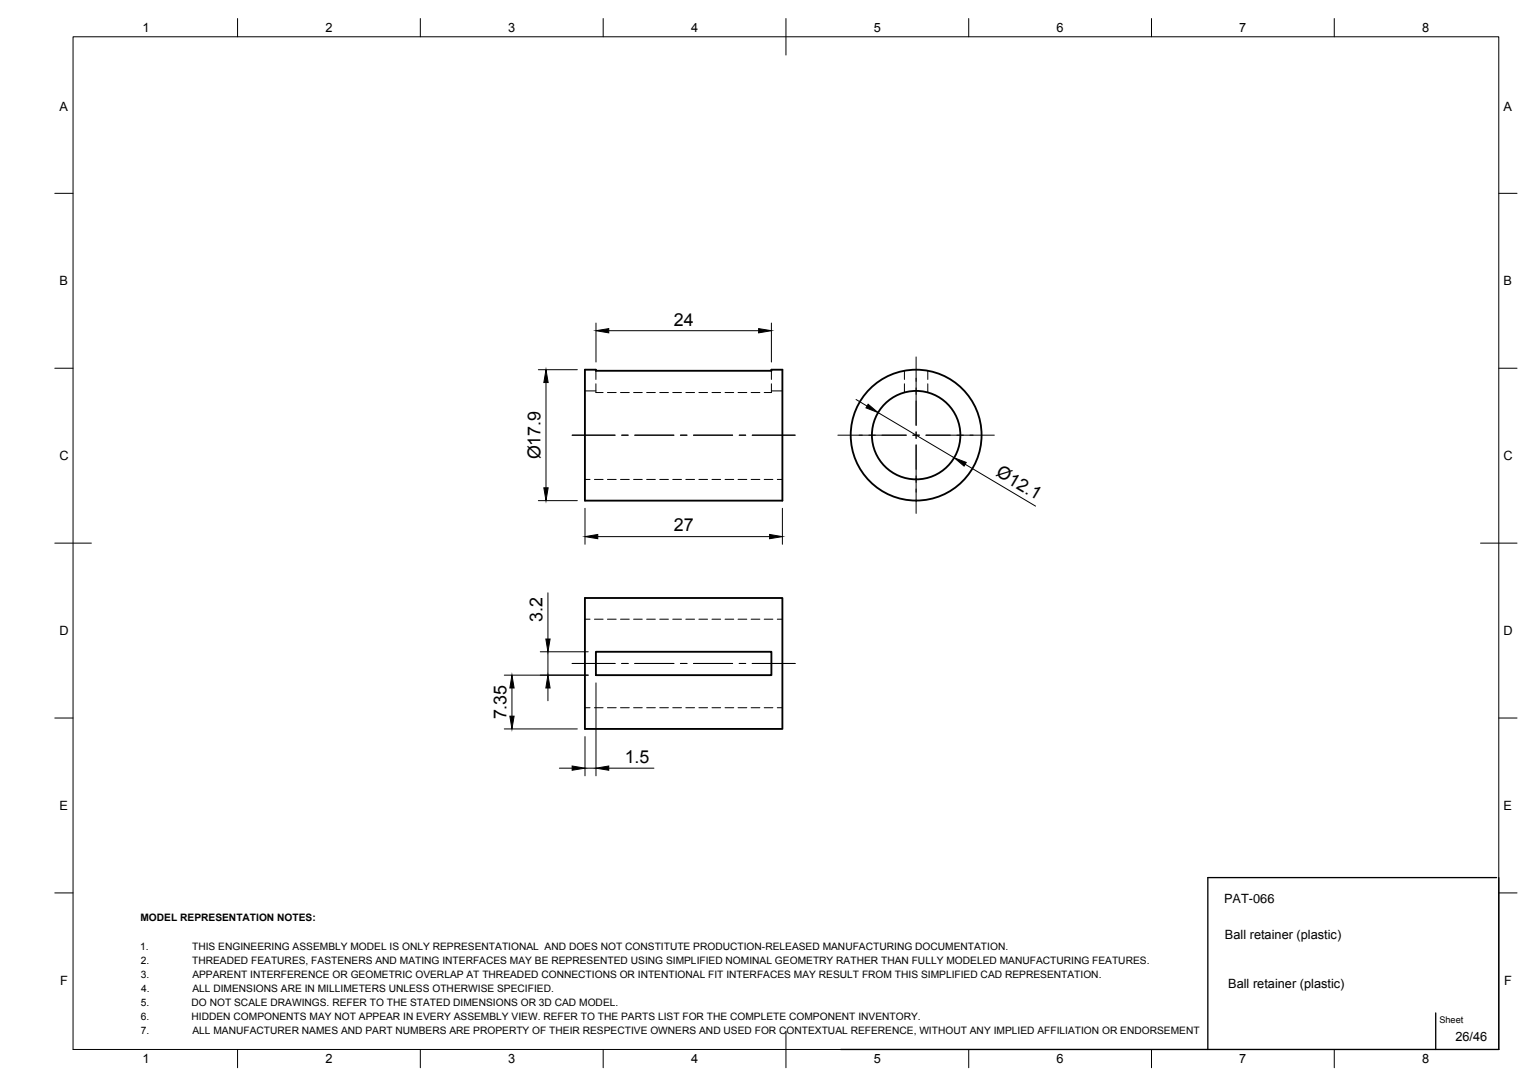
ISO-10303-21;
HEADER;
/* Generated by software containing ST-Developer
 * from STEP Tools, Inc. (www.steptools.com) 
 */

FILE_DESCRIPTION(
/* description */ ('Lever-operated bar clamp (toggle)'),
/* implementation_level */ '2;1');

FILE_NAME(
/* name */ 'Ball retainer (plastic).step',
/* time_stamp */ '2026-10-28T03:25:02-07:00',
/* author */ (''),
/* organization */ (''),
/* preprocessor_version */ 'ST-DEVELOPER v20.2',
/* originating_system */ 'Autodesk Translation Framework v15.17.0.0',
/* authorisation */ '');

FILE_SCHEMA (('AUTOMOTIVE_DESIGN { 1 0 10303 214 3 1 1 }'));
ENDSEC;

DATA;
#10=MECHANICAL_DESIGN_GEOMETRIC_PRESENTATION_REPRESENTATION('',(#436),#12413);
#352=SHAPE_REPRESENTATION_RELATIONSHIP('SRR','None',#12593,#390);
#390=ADVANCED_BREP_SHAPE_REPRESENTATION('',(#482),#12390);
#436=STYLED_ITEM('',(#12862),#482);
#482=MANIFOLD_SOLID_BREP('Body1',#6596);
#604=FACE_BOUND('',#1622,.T.);
#605=FACE_BOUND('',#1624,.T.);
#606=FACE_BOUND('',#1626,.T.);
#607=FACE_BOUND('',#1628,.T.);
#767=PLANE('',#7495);
#768=PLANE('',#7498);
#769=PLANE('',#7499);
#770=PLANE('',#7502);
#771=PLANE('',#7503);
#772=PLANE('',#7508);
#1107=FACE_OUTER_BOUND('',#1617,.T.);
#1108=FACE_OUTER_BOUND('',#1618,.T.);
#1109=FACE_OUTER_BOUND('',#1619,.T.);
#1110=FACE_OUTER_BOUND('',#1620,.T.);
#1111=FACE_OUTER_BOUND('',#1621,.T.);
#1112=FACE_OUTER_BOUND('',#1623,.T.);
#1113=FACE_OUTER_BOUND('',#1625,.T.);
#1114=FACE_OUTER_BOUND('',#1627,.T.);
#1617=EDGE_LOOP('',(#5317,#5318,#5319,#5320));
#1618=EDGE_LOOP('',(#5321,#5322,#5323,#5324));
#1619=EDGE_LOOP('',(#5325,#5326,#5327,#5328));
#1620=EDGE_LOOP('',(#5329,#5330,#5331,#5332));
#1621=EDGE_LOOP('',(#5333));
#1622=EDGE_LOOP('',(#5334));
#1623=EDGE_LOOP('',(#5335,#5336,#5337,#5338));
#1624=EDGE_LOOP('',(#5339,#5340,#5341,#5342));
#1625=EDGE_LOOP('',(#5343));
#1626=EDGE_LOOP('',(#5344));
#1627=EDGE_LOOP('',(#5345,#5346,#5347,#5348));
#1628=EDGE_LOOP('',(#5349,#5350,#5351,#5352));
#2072=LINE('',#11390,#2513);
#2073=LINE('',#11393,#2514);
#2074=LINE('',#11396,#2515);
#2075=LINE('',#11398,#2516);
#2076=LINE('',#11399,#2517);
#2077=LINE('',#11405,#2518);
#2078=LINE('',#11407,#2519);
#2079=LINE('',#11408,#2520);
#2080=LINE('',#11417,#2521);
#2081=LINE('',#11422,#2522);
#2513=VECTOR('',#9031,1.);
#2514=VECTOR('',#9034,1.);
#2515=VECTOR('',#9037,1.);
#2516=VECTOR('',#9038,1.);
#2517=VECTOR('',#9039,1.);
#2518=VECTOR('',#9046,1.);
#2519=VECTOR('',#9049,1.);
#2520=VECTOR('',#9050,1.);
#2521=VECTOR('',#9061,0.895);
#2522=VECTOR('',#9068,0.605);
#2942=CIRCLE('',#7496,0.895);
#2943=CIRCLE('',#7497,0.605);
#2944=CIRCLE('',#7500,0.895);
#2945=CIRCLE('',#7501,0.605);
#2946=CIRCLE('',#7504,0.895);
#2947=CIRCLE('',#7505,0.605);
#2948=CIRCLE('',#7507,0.895);
#2949=CIRCLE('',#7509,0.605);
#3381=VERTEX_POINT('',#11386);
#3382=VERTEX_POINT('',#11387);
#3383=VERTEX_POINT('',#11389);
#3384=VERTEX_POINT('',#11391);
#3385=VERTEX_POINT('',#11395);
#3386=VERTEX_POINT('',#11397);
#3387=VERTEX_POINT('',#11401);
#3388=VERTEX_POINT('',#11403);
#3389=VERTEX_POINT('',#11410);
#3390=VERTEX_POINT('',#11412);
#3391=VERTEX_POINT('',#11415);
#3392=VERTEX_POINT('',#11419);
#4063=EDGE_CURVE('',#3381,#3382,#2942,.T.);
#4064=EDGE_CURVE('',#3383,#3381,#2072,.T.);
#4065=EDGE_CURVE('',#3384,#3383,#2943,.T.);
#4066=EDGE_CURVE('',#3382,#3384,#2073,.T.);
#4067=EDGE_CURVE('',#3382,#3385,#2074,.T.);
#4068=EDGE_CURVE('',#3386,#3384,#2075,.T.);
#4069=EDGE_CURVE('',#3386,#3385,#2076,.T.);
#4070=EDGE_CURVE('',#3385,#3387,#2944,.T.);
#4071=EDGE_CURVE('',#3388,#3386,#2945,.T.);
#4072=EDGE_CURVE('',#3387,#3388,#2077,.T.);
#4073=EDGE_CURVE('',#3387,#3381,#2078,.T.);
#4074=EDGE_CURVE('',#3383,#3388,#2079,.T.);
#4075=EDGE_CURVE('',#3389,#3389,#2946,.T.);
#4076=EDGE_CURVE('',#3390,#3390,#2947,.T.);
#4077=EDGE_CURVE('',#3391,#3391,#2948,.T.);
#4078=EDGE_CURVE('',#3391,#3389,#2080,.T.);
#4079=EDGE_CURVE('',#3392,#3392,#2949,.T.);
#4080=EDGE_CURVE('',#3392,#3390,#2081,.T.);
#5317=ORIENTED_EDGE('',*,*,#4063,.F.);
#5318=ORIENTED_EDGE('',*,*,#4064,.F.);
#5319=ORIENTED_EDGE('',*,*,#4065,.F.);
#5320=ORIENTED_EDGE('',*,*,#4066,.F.);
#5321=ORIENTED_EDGE('',*,*,#4067,.F.);
#5322=ORIENTED_EDGE('',*,*,#4066,.T.);
#5323=ORIENTED_EDGE('',*,*,#4068,.F.);
#5324=ORIENTED_EDGE('',*,*,#4069,.T.);
#5325=ORIENTED_EDGE('',*,*,#4070,.F.);
#5326=ORIENTED_EDGE('',*,*,#4069,.F.);
#5327=ORIENTED_EDGE('',*,*,#4071,.F.);
#5328=ORIENTED_EDGE('',*,*,#4072,.F.);
#5329=ORIENTED_EDGE('',*,*,#4073,.F.);
#5330=ORIENTED_EDGE('',*,*,#4072,.T.);
#5331=ORIENTED_EDGE('',*,*,#4074,.F.);
#5332=ORIENTED_EDGE('',*,*,#4064,.T.);
#5333=ORIENTED_EDGE('',*,*,#4075,.F.);
#5334=ORIENTED_EDGE('',*,*,#4076,.T.);
#5335=ORIENTED_EDGE('',*,*,#4077,.F.);
#5336=ORIENTED_EDGE('',*,*,#4078,.T.);
#5337=ORIENTED_EDGE('',*,*,#4075,.T.);
#5338=ORIENTED_EDGE('',*,*,#4078,.F.);
#5339=ORIENTED_EDGE('',*,*,#4070,.T.);
#5340=ORIENTED_EDGE('',*,*,#4073,.T.);
#5341=ORIENTED_EDGE('',*,*,#4063,.T.);
#5342=ORIENTED_EDGE('',*,*,#4067,.T.);
#5343=ORIENTED_EDGE('',*,*,#4077,.T.);
#5344=ORIENTED_EDGE('',*,*,#4079,.F.);
#5345=ORIENTED_EDGE('',*,*,#4079,.T.);
#5346=ORIENTED_EDGE('',*,*,#4080,.T.);
#5347=ORIENTED_EDGE('',*,*,#4076,.F.);
#5348=ORIENTED_EDGE('',*,*,#4080,.F.);
#5349=ORIENTED_EDGE('',*,*,#4071,.T.);
#5350=ORIENTED_EDGE('',*,*,#4068,.T.);
#5351=ORIENTED_EDGE('',*,*,#4065,.T.);
#5352=ORIENTED_EDGE('',*,*,#4074,.T.);
#6111=CYLINDRICAL_SURFACE('',#7506,0.895);
#6112=CYLINDRICAL_SURFACE('',#7510,0.605);
#6382=ADVANCED_FACE('',(#1107),#767,.F.);
#6383=ADVANCED_FACE('',(#1108),#768,.F.);
#6384=ADVANCED_FACE('',(#1109),#769,.F.);
#6385=ADVANCED_FACE('',(#1110),#770,.F.);
#6386=ADVANCED_FACE('',(#1111,#604),#771,.T.);
#6387=ADVANCED_FACE('',(#1112,#605),#6111,.T.);
#6388=ADVANCED_FACE('',(#1113,#606),#772,.T.);
#6389=ADVANCED_FACE('',(#1114,#607),#6112,.F.);
#6596=CLOSED_SHELL('',(#6382,#6383,#6384,#6385,#6386,#6387,#6388,#6389));
#7494=AXIS2_PLACEMENT_3D('',#11384,#9025,#9026);
#7495=AXIS2_PLACEMENT_3D('',#11385,#9027,#9028);
#7496=AXIS2_PLACEMENT_3D('',#11388,#9029,#9030);
#7497=AXIS2_PLACEMENT_3D('',#11392,#9032,#9033);
#7498=AXIS2_PLACEMENT_3D('',#11394,#9035,#9036);
#7499=AXIS2_PLACEMENT_3D('',#11400,#9040,#9041);
#7500=AXIS2_PLACEMENT_3D('',#11402,#9042,#9043);
#7501=AXIS2_PLACEMENT_3D('',#11404,#9044,#9045);
#7502=AXIS2_PLACEMENT_3D('',#11406,#9047,#9048);
#7503=AXIS2_PLACEMENT_3D('',#11409,#9051,#9052);
#7504=AXIS2_PLACEMENT_3D('',#11411,#9053,#9054);
#7505=AXIS2_PLACEMENT_3D('',#11413,#9055,#9056);
#7506=AXIS2_PLACEMENT_3D('',#11414,#9057,#9058);
#7507=AXIS2_PLACEMENT_3D('',#11416,#9059,#9060);
#7508=AXIS2_PLACEMENT_3D('',#11418,#9062,#9063);
#7509=AXIS2_PLACEMENT_3D('',#11420,#9064,#9065);
#7510=AXIS2_PLACEMENT_3D('',#11421,#9066,#9067);
#9025=DIRECTION('axis',(0.,0.,1.));
#9026=DIRECTION('refdir',(1.,0.,0.));
#9027=DIRECTION('center_axis',(0.,1.,0.));
#9028=DIRECTION('ref_axis',(0.,0.,1.));
#9029=DIRECTION('center_axis',(0.,1.,0.));
#9030=DIRECTION('ref_axis',(1.,0.,0.));
#9031=DIRECTION('',(1.,0.,0.));
#9032=DIRECTION('center_axis',(0.,-1.,0.));
#9033=DIRECTION('ref_axis',(1.,0.,0.));
#9034=DIRECTION('',(-1.,0.,0.));
#9035=DIRECTION('center_axis',(0.,0.,-1.));
#9036=DIRECTION('ref_axis',(-1.,0.,0.));
#9037=DIRECTION('',(0.,-1.,0.));
#9038=DIRECTION('',(0.,1.,0.));
#9039=DIRECTION('',(1.,0.,0.));
#9040=DIRECTION('center_axis',(0.,-1.,0.));
#9041=DIRECTION('ref_axis',(0.,0.,-1.));
#9042=DIRECTION('center_axis',(0.,-1.,0.));
#9043=DIRECTION('ref_axis',(1.,0.,0.));
#9044=DIRECTION('center_axis',(0.,1.,0.));
#9045=DIRECTION('ref_axis',(1.,0.,0.));
#9046=DIRECTION('',(-1.,0.,0.));
#9047=DIRECTION('center_axis',(0.,0.,1.));
#9048=DIRECTION('ref_axis',(1.,0.,0.));
#9049=DIRECTION('',(0.,1.,0.));
#9050=DIRECTION('',(0.,-1.,0.));
#9051=DIRECTION('center_axis',(0.,1.,0.));
#9052=DIRECTION('ref_axis',(0.,0.,1.));
#9053=DIRECTION('center_axis',(0.,-1.,0.));
#9054=DIRECTION('ref_axis',(1.,0.,0.));
#9055=DIRECTION('center_axis',(0.,-1.,0.));
#9056=DIRECTION('ref_axis',(1.,0.,0.));
#9057=DIRECTION('center_axis',(0.,-1.,0.));
#9058=DIRECTION('ref_axis',(1.,0.,0.));
#9059=DIRECTION('center_axis',(0.,-1.,0.));
#9060=DIRECTION('ref_axis',(1.,0.,0.));
#9061=DIRECTION('',(0.,1.,0.));
#9062=DIRECTION('center_axis',(0.,-1.,0.));
#9063=DIRECTION('ref_axis',(0.,0.,-1.));
#9064=DIRECTION('center_axis',(0.,-1.,0.));
#9065=DIRECTION('ref_axis',(1.,0.,0.));
#9066=DIRECTION('center_axis',(0.,-1.,0.));
#9067=DIRECTION('ref_axis',(1.,0.,0.));
#9068=DIRECTION('',(0.,1.,0.));
#11384=CARTESIAN_POINT('',(0.,0.,0.));
#11385=CARTESIAN_POINT('Origin',(0.75,1.2,0.));
#11386=CARTESIAN_POINT('',(0.880582193778639,1.2,0.16));
#11387=CARTESIAN_POINT('',(0.880582193778639,1.2,-0.16));
#11388=CARTESIAN_POINT('Origin',(0.,1.2,0.));
#11389=CARTESIAN_POINT('',(0.583459510163302,1.2,0.16));
#11390=CARTESIAN_POINT('',(0.57,1.2,0.16));
#11391=CARTESIAN_POINT('',(0.583459510163302,1.2,-0.16));
#11392=CARTESIAN_POINT('Origin',(0.,1.2,0.));
#11393=CARTESIAN_POINT('',(0.93,1.2,-0.16));
#11394=CARTESIAN_POINT('Origin',(0.93,0.,-0.16));
#11395=CARTESIAN_POINT('',(0.880582193778639,-1.2,-0.16));
#11396=CARTESIAN_POINT('',(0.880582193778639,0.,-0.16));
#11397=CARTESIAN_POINT('',(0.583459510163302,-1.2,-0.16));
#11398=CARTESIAN_POINT('',(0.583459510163302,0.,-0.16));
#11399=CARTESIAN_POINT('',(0.93,-1.2,-0.16));
#11400=CARTESIAN_POINT('Origin',(0.75,-1.2,0.));
#11401=CARTESIAN_POINT('',(0.880582193778639,-1.2,0.16));
#11402=CARTESIAN_POINT('Origin',(0.,-1.2,0.));
#11403=CARTESIAN_POINT('',(0.583459510163302,-1.2,0.16));
#11404=CARTESIAN_POINT('Origin',(0.,-1.2,0.));
#11405=CARTESIAN_POINT('',(0.57,-1.2,0.16));
#11406=CARTESIAN_POINT('Origin',(0.57,0.,0.16));
#11407=CARTESIAN_POINT('',(0.880582193778639,0.,0.16));
#11408=CARTESIAN_POINT('',(0.583459510163302,0.,0.16));
#11409=CARTESIAN_POINT('Origin',(0.895,1.35,0.));
#11410=CARTESIAN_POINT('',(-0.895,1.35,-1.09605888523688E-16));
#11411=CARTESIAN_POINT('Origin',(0.,1.35,0.));
#11412=CARTESIAN_POINT('',(-0.605,1.35,-7.40911313484149E-17));
#11413=CARTESIAN_POINT('Origin',(0.,1.35,0.));
#11414=CARTESIAN_POINT('Origin',(0.,0.,0.));
#11415=CARTESIAN_POINT('',(-0.895,-1.35,-1.09605888523688E-16));
#11416=CARTESIAN_POINT('Origin',(0.,-1.35,0.));
#11417=CARTESIAN_POINT('',(-0.895,0.,-1.09605888523688E-16));
#11418=CARTESIAN_POINT('Origin',(0.605,-1.35,0.));
#11419=CARTESIAN_POINT('',(-0.605,-1.35,-7.40911313484149E-17));
#11420=CARTESIAN_POINT('Origin',(0.,-1.35,0.));
#11421=CARTESIAN_POINT('Origin',(0.,0.,0.));
#11422=CARTESIAN_POINT('',(-0.605,0.,-7.40911313484149E-17));
#12344=UNCERTAINTY_MEASURE_WITH_UNIT(LENGTH_MEASURE(0.001),#12414,
'DISTANCE_ACCURACY_VALUE',
'Maximum model space distance between geometric entities at asserted c
onnectivities');
#12367=UNCERTAINTY_MEASURE_WITH_UNIT(LENGTH_MEASURE(0.001),#12414,
'DISTANCE_ACCURACY_VALUE',
'Maximum model space distance between geometric entities at asserted c
onnectivities');
#12390=(
GEOMETRIC_REPRESENTATION_CONTEXT(3)
GLOBAL_UNCERTAINTY_ASSIGNED_CONTEXT((#12344))
GLOBAL_UNIT_ASSIGNED_CONTEXT((#12414,#12416,#12417))
REPRESENTATION_CONTEXT('','3D')
);
#12413=(
GEOMETRIC_REPRESENTATION_CONTEXT(3)
GLOBAL_UNCERTAINTY_ASSIGNED_CONTEXT((#12367))
GLOBAL_UNIT_ASSIGNED_CONTEXT((#12414,#12416,#12417))
REPRESENTATION_CONTEXT('','3D')
);
#12414=(
LENGTH_UNIT()
NAMED_UNIT(*)
SI_UNIT(.CENTI.,.METRE.)
);
#12416=(
NAMED_UNIT(*)
PLANE_ANGLE_UNIT()
SI_UNIT($,.RADIAN.)
);
#12417=(
NAMED_UNIT(*)
SI_UNIT($,.STERADIAN.)
SOLID_ANGLE_UNIT()
);
#12440=SHAPE_DEFINITION_REPRESENTATION(#12490,#12593);
#12490=PRODUCT_DEFINITION_SHAPE('',$,#12639);
#12593=SHAPE_REPRESENTATION('',(#7494),#12390);
#12616=PRODUCT_DEFINITION_CONTEXT('part definition',#12753,'design');
#12639=PRODUCT_DEFINITION('Ball retainer (plastic)',
'Ball retainer (plastic)',#12684,#12616);
#12684=PRODUCT_DEFINITION_FORMATION('',$,#12777);
#12753=APPLICATION_CONTEXT(
'Core Data for Automotive Mechanical Design Process');
#12754=PRODUCT_CONTEXT('part definition',#12753,'mechanical');
#12777=PRODUCT('Ball retainer (plastic)','Ball retainer (plastic)',
'Ball retainer (plastic)',(#12754));
#12856=COLOUR_RGB('Sky Blue',0.24,0.69,0.87);
#12857=FILL_AREA_STYLE_COLOUR('',#12856);
#12858=FILL_AREA_STYLE('',(#12857));
#12859=SURFACE_STYLE_FILL_AREA(#12858);
#12860=SURFACE_SIDE_STYLE('',(#12859));
#12861=SURFACE_STYLE_USAGE(.BOTH.,#12860);
#12862=PRESENTATION_STYLE_ASSIGNMENT((#12861));
ENDSEC;
END-ISO-10303-21;
